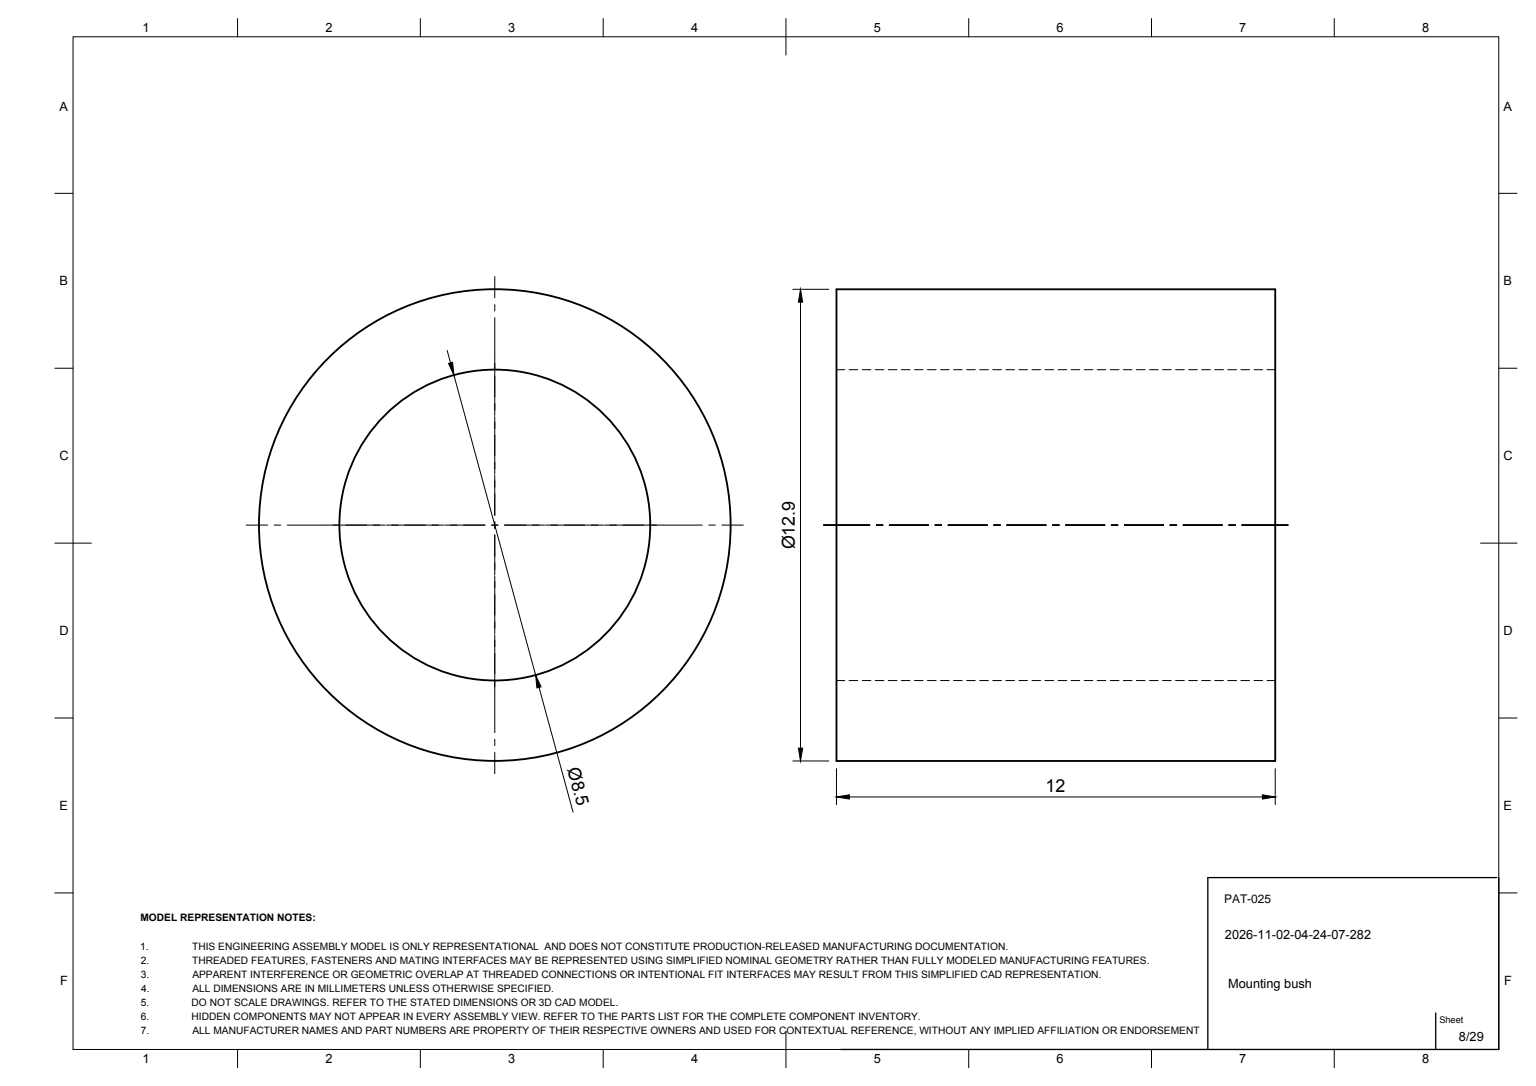
ISO-10303-21;
HEADER;
/* Generated by software containing ST-Developer
 * from STEP Tools, Inc. (www.steptools.com) 
 */

FILE_DESCRIPTION(
/* description */ ('Counter shaft with two pulleys and keyed hub'),
/* implementation_level */ '2;1');

FILE_NAME(
/* name */ 'Mounting bush.step',
/* time_stamp */ '2026-10-27T10:46:10-07:00',
/* author */ (''),
/* organization */ (''),
/* preprocessor_version */ 'ST-DEVELOPER v20.2',
/* originating_system */ 'Autodesk Translation Framework v15.17.0.0',
/* authorisation */ '');

FILE_SCHEMA (('AUTOMOTIVE_DESIGN { 1 0 10303 214 3 1 1 }'));
ENDSEC;

DATA;
#10=MECHANICAL_DESIGN_GEOMETRIC_PRESENTATION_REPRESENTATION('',(#293),#10821);
#243=SHAPE_REPRESENTATION_RELATIONSHIP('SRR','None',#10929,#268);
#268=ADVANCED_BREP_SHAPE_REPRESENTATION('',(#319),#10797);
#293=STYLED_ITEM('',(#11128),#319);
#319=MANIFOLD_SOLID_BREP('Body1',#5576);
#348=FACE_BOUND('',#935,.T.);
#349=FACE_BOUND('',#937,.T.);
#449=PLANE('',#5919);
#450=PLANE('',#5920);
#610=FACE_OUTER_BOUND('',#932,.T.);
#611=FACE_OUTER_BOUND('',#933,.T.);
#612=FACE_OUTER_BOUND('',#934,.T.);
#613=FACE_OUTER_BOUND('',#936,.T.);
#932=EDGE_LOOP('',(#3725,#3726,#3727,#3728));
#933=EDGE_LOOP('',(#3729,#3730,#3731,#3732));
#934=EDGE_LOOP('',(#3733));
#935=EDGE_LOOP('',(#3734));
#936=EDGE_LOOP('',(#3735));
#937=EDGE_LOOP('',(#3736));
#1347=LINE('',#8424,#1736);
#1348=LINE('',#8430,#1737);
#1736=VECTOR('',#6675,0.425);
#1737=VECTOR('',#6682,0.645);
#2093=CIRCLE('',#5914,0.425);
#2094=CIRCLE('',#5915,0.425);
#2095=CIRCLE('',#5917,0.645);
#2096=CIRCLE('',#5918,0.645);
#2416=VERTEX_POINT('',#8421);
#2417=VERTEX_POINT('',#8423);
#2418=VERTEX_POINT('',#8427);
#2419=VERTEX_POINT('',#8429);
#2935=EDGE_CURVE('',#2416,#2416,#2093,.T.);
#2936=EDGE_CURVE('',#2416,#2417,#1347,.T.);
#2937=EDGE_CURVE('',#2417,#2417,#2094,.T.);
#2938=EDGE_CURVE('',#2418,#2418,#2095,.T.);
#2939=EDGE_CURVE('',#2418,#2419,#1348,.T.);
#2940=EDGE_CURVE('',#2419,#2419,#2096,.T.);
#3725=ORIENTED_EDGE('',*,*,#2935,.F.);
#3726=ORIENTED_EDGE('',*,*,#2936,.T.);
#3727=ORIENTED_EDGE('',*,*,#2937,.T.);
#3728=ORIENTED_EDGE('',*,*,#2936,.F.);
#3729=ORIENTED_EDGE('',*,*,#2938,.F.);
#3730=ORIENTED_EDGE('',*,*,#2939,.T.);
#3731=ORIENTED_EDGE('',*,*,#2940,.T.);
#3732=ORIENTED_EDGE('',*,*,#2939,.F.);
#3733=ORIENTED_EDGE('',*,*,#2938,.T.);
#3734=ORIENTED_EDGE('',*,*,#2935,.T.);
#3735=ORIENTED_EDGE('',*,*,#2940,.F.);
#3736=ORIENTED_EDGE('',*,*,#2937,.F.);
#5117=CYLINDRICAL_SURFACE('',#5913,0.425);
#5118=CYLINDRICAL_SURFACE('',#5916,0.645);
#5281=ADVANCED_FACE('',(#610),#5117,.F.);
#5282=ADVANCED_FACE('',(#611),#5118,.T.);
#5283=ADVANCED_FACE('',(#612,#348),#449,.T.);
#5284=ADVANCED_FACE('',(#613,#349),#450,.F.);
#5576=CLOSED_SHELL('',(#5281,#5282,#5283,#5284));
#5912=AXIS2_PLACEMENT_3D('',#8419,#6669,#6670);
#5913=AXIS2_PLACEMENT_3D('',#8420,#6671,#6672);
#5914=AXIS2_PLACEMENT_3D('',#8422,#6673,#6674);
#5915=AXIS2_PLACEMENT_3D('',#8425,#6676,#6677);
#5916=AXIS2_PLACEMENT_3D('',#8426,#6678,#6679);
#5917=AXIS2_PLACEMENT_3D('',#8428,#6680,#6681);
#5918=AXIS2_PLACEMENT_3D('',#8431,#6683,#6684);
#5919=AXIS2_PLACEMENT_3D('',#8432,#6685,#6686);
#5920=AXIS2_PLACEMENT_3D('',#8433,#6687,#6688);
#6669=DIRECTION('axis',(0.,0.,1.));
#6670=DIRECTION('refdir',(1.,0.,0.));
#6671=DIRECTION('center_axis',(0.,0.,1.));
#6672=DIRECTION('ref_axis',(1.,0.,0.));
#6673=DIRECTION('center_axis',(0.,0.,-1.));
#6674=DIRECTION('ref_axis',(1.,0.,0.));
#6675=DIRECTION('',(0.,0.,-1.));
#6676=DIRECTION('center_axis',(0.,0.,-1.));
#6677=DIRECTION('ref_axis',(1.,0.,0.));
#6678=DIRECTION('center_axis',(0.,0.,1.));
#6679=DIRECTION('ref_axis',(1.,0.,0.));
#6680=DIRECTION('center_axis',(0.,0.,1.));
#6681=DIRECTION('ref_axis',(1.,0.,0.));
#6682=DIRECTION('',(0.,0.,-1.));
#6683=DIRECTION('center_axis',(0.,0.,1.));
#6684=DIRECTION('ref_axis',(1.,0.,0.));
#6685=DIRECTION('center_axis',(0.,0.,1.));
#6686=DIRECTION('ref_axis',(1.,0.,0.));
#6687=DIRECTION('center_axis',(0.,0.,1.));
#6688=DIRECTION('ref_axis',(1.,0.,0.));
#8419=CARTESIAN_POINT('',(0.,0.,0.));
#8420=CARTESIAN_POINT('Origin',(-4.75,0.,1.2));
#8421=CARTESIAN_POINT('',(-5.175,-5.20474889637625E-17,2.4));
#8422=CARTESIAN_POINT('Origin',(-4.75,0.,2.4));
#8423=CARTESIAN_POINT('',(-5.175,-5.20474889637625E-17,1.2));
#8424=CARTESIAN_POINT('',(-5.175,-5.20474889637625E-17,1.2));
#8425=CARTESIAN_POINT('Origin',(-4.75,0.,1.2));
#8426=CARTESIAN_POINT('Origin',(-4.75,0.,1.2));
#8427=CARTESIAN_POINT('',(-5.395,-7.89897185450042E-17,2.4));
#8428=CARTESIAN_POINT('Origin',(-4.75,0.,2.4));
#8429=CARTESIAN_POINT('',(-5.395,-7.89897185450042E-17,1.2));
#8430=CARTESIAN_POINT('',(-5.395,-7.89897185450042E-17,1.2));
#8431=CARTESIAN_POINT('Origin',(-4.75,0.,1.2));
#8432=CARTESIAN_POINT('Origin',(-4.75,0.,2.4));
#8433=CARTESIAN_POINT('Origin',(-4.75,0.,1.2));
#10767=UNCERTAINTY_MEASURE_WITH_UNIT(LENGTH_MEASURE(0.001),#10822,
'DISTANCE_ACCURACY_VALUE',
'Maximum model space distance between geometric entities at asserted c
onnectivities');
#10791=UNCERTAINTY_MEASURE_WITH_UNIT(LENGTH_MEASURE(0.001),#10822,
'DISTANCE_ACCURACY_VALUE',
'Maximum model space distance between geometric entities at asserted c
onnectivities');
#10797=(
GEOMETRIC_REPRESENTATION_CONTEXT(3)
GLOBAL_UNCERTAINTY_ASSIGNED_CONTEXT((#10767))
GLOBAL_UNIT_ASSIGNED_CONTEXT((#10822,#10824,#10825))
REPRESENTATION_CONTEXT('','3D')
);
#10821=(
GEOMETRIC_REPRESENTATION_CONTEXT(3)
GLOBAL_UNCERTAINTY_ASSIGNED_CONTEXT((#10791))
GLOBAL_UNIT_ASSIGNED_CONTEXT((#10822,#10824,#10825))
REPRESENTATION_CONTEXT('','3D')
);
#10822=(
LENGTH_UNIT()
NAMED_UNIT(*)
SI_UNIT(.CENTI.,.METRE.)
);
#10824=(
NAMED_UNIT(*)
PLANE_ANGLE_UNIT()
SI_UNIT($,.RADIAN.)
);
#10825=(
NAMED_UNIT(*)
SI_UNIT($,.STERADIAN.)
SOLID_ANGLE_UNIT()
);
#10831=SHAPE_DEFINITION_REPRESENTATION(#10860,#10929);
#10860=PRODUCT_DEFINITION_SHAPE('',$,#10959);
#10929=SHAPE_REPRESENTATION('',(#5912),#10797);
#10953=PRODUCT_DEFINITION_CONTEXT('part definition',#11042,'design');
#10959=PRODUCT_DEFINITION('Mounting bush','Mounting bush',#10988,#10953);
#10988=PRODUCT_DEFINITION_FORMATION('',$,#11049);
#11042=APPLICATION_CONTEXT(
'Core Data for Automotive Mechanical Design Process');
#11043=PRODUCT_CONTEXT('part definition',#11042,'mechanical');
#11049=PRODUCT('Mounting bush','Mounting bush','Mounting bush',(#11043));
#11122=COLOUR_RGB('Sky Blue',0.24,0.69,0.87);
#11123=FILL_AREA_STYLE_COLOUR('',#11122);
#11124=FILL_AREA_STYLE('',(#11123));
#11125=SURFACE_STYLE_FILL_AREA(#11124);
#11126=SURFACE_SIDE_STYLE('',(#11125));
#11127=SURFACE_STYLE_USAGE(.BOTH.,#11126);
#11128=PRESENTATION_STYLE_ASSIGNMENT((#11127));
ENDSEC;
END-ISO-10303-21;
